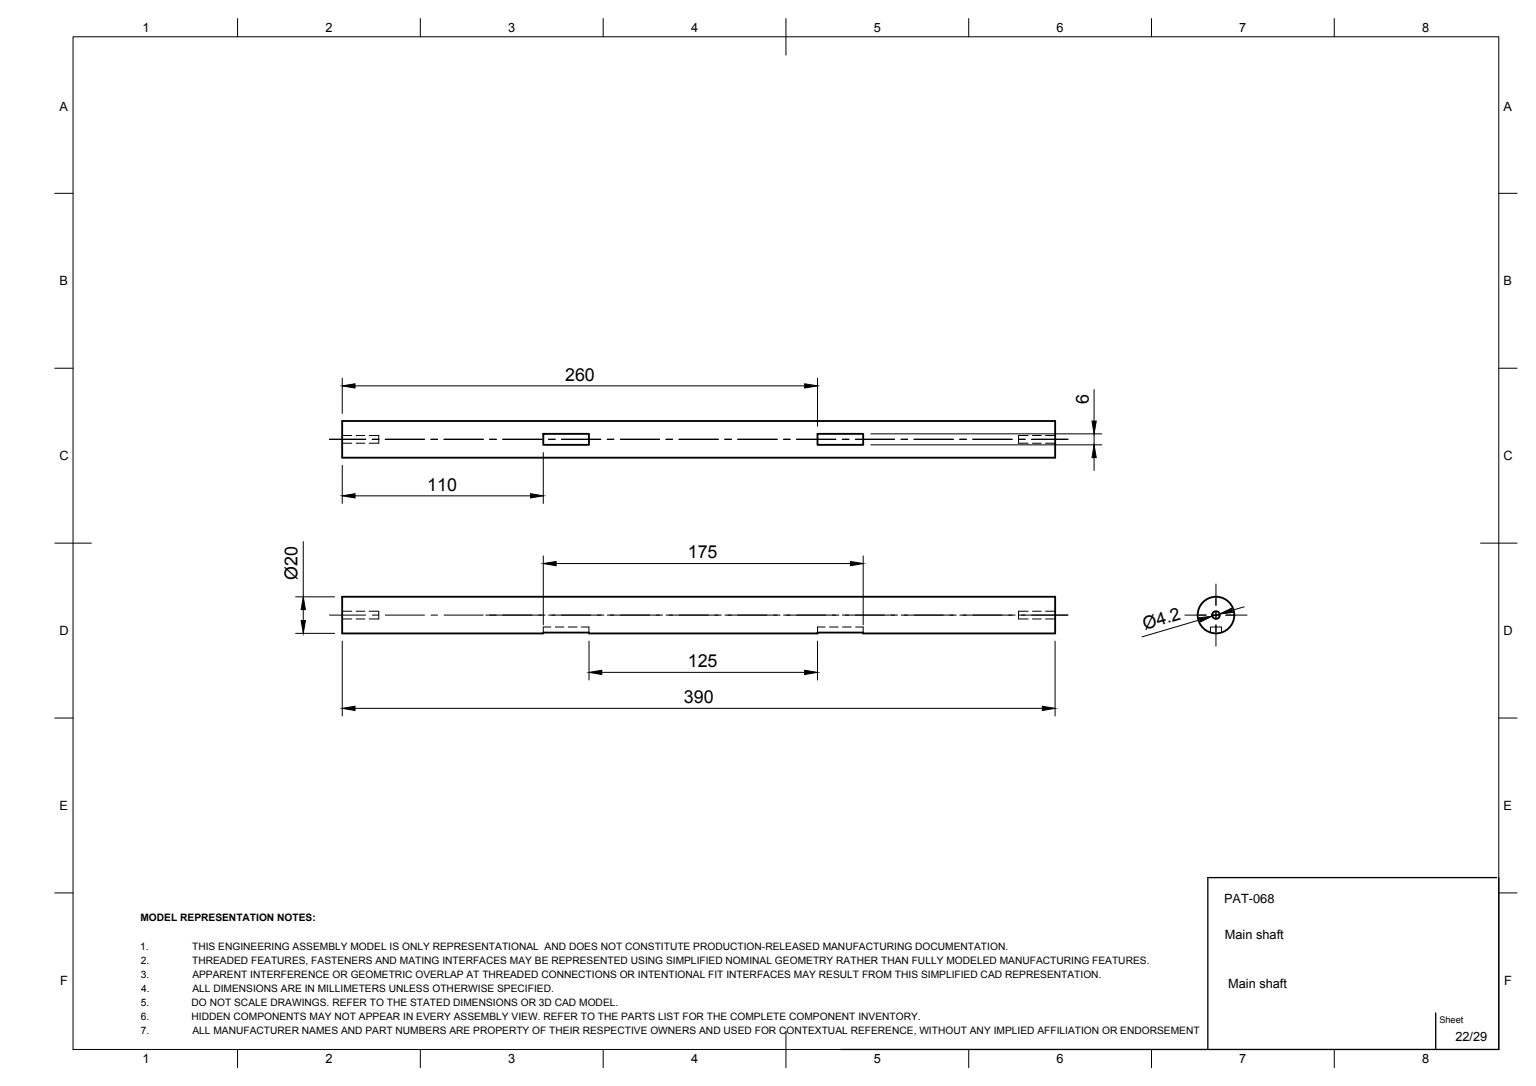
ISO-10303-21;
HEADER;
/* Generated by software containing ST-Developer
 * from STEP Tools, Inc. (www.steptools.com) 
 */

FILE_DESCRIPTION(
/* description */ ('Line shaft on three pillow blocks'),
/* implementation_level */ '2;1');

FILE_NAME(
/* name */ 'Main shaft.step',
/* time_stamp */ '2026-10-27T10:49:19-07:00',
/* author */ (''),
/* organization */ (''),
/* preprocessor_version */ 'ST-DEVELOPER v20.2',
/* originating_system */ 'Autodesk Translation Framework v15.17.0.0',
/* authorisation */ '');

FILE_SCHEMA (('AUTOMOTIVE_DESIGN { 1 0 10303 214 3 1 1 }'));
ENDSEC;

DATA;
#10=MECHANICAL_DESIGN_GEOMETRIC_PRESENTATION_REPRESENTATION('',(#356),#8377);
#301=SHAPE_REPRESENTATION_RELATIONSHIP('SRR','None',#8518,#328);
#328=ADVANCED_BREP_SHAPE_REPRESENTATION('',(#382),#8367);
#356=STYLED_ITEM('',(#8718),#382);
#382=MANIFOLD_SOLID_BREP('Body1',#4344);
#462=FACE_BOUND('',#1146,.T.);
#463=FACE_BOUND('',#1147,.T.);
#464=FACE_BOUND('',#1149,.T.);
#465=FACE_BOUND('',#1151,.T.);
#584=PLANE('',#4969);
#585=PLANE('',#4973);
#586=PLANE('',#4974);
#587=PLANE('',#4975);
#588=PLANE('',#4977);
#589=PLANE('',#4978);
#590=PLANE('',#4979);
#591=PLANE('',#4981);
#592=PLANE('',#4982);
#593=PLANE('',#4984);
#594=PLANE('',#4985);
#595=PLANE('',#4986);
#596=PLANE('',#4991);
#597=PLANE('',#4992);
#808=FACE_OUTER_BOUND('',#1131,.T.);
#809=FACE_OUTER_BOUND('',#1132,.T.);
#810=FACE_OUTER_BOUND('',#1133,.T.);
#811=FACE_OUTER_BOUND('',#1134,.T.);
#812=FACE_OUTER_BOUND('',#1135,.T.);
#813=FACE_OUTER_BOUND('',#1136,.T.);
#814=FACE_OUTER_BOUND('',#1137,.T.);
#815=FACE_OUTER_BOUND('',#1138,.T.);
#816=FACE_OUTER_BOUND('',#1139,.T.);
#817=FACE_OUTER_BOUND('',#1140,.T.);
#818=FACE_OUTER_BOUND('',#1141,.T.);
#819=FACE_OUTER_BOUND('',#1142,.T.);
#820=FACE_OUTER_BOUND('',#1143,.T.);
#821=FACE_OUTER_BOUND('',#1144,.T.);
#822=FACE_OUTER_BOUND('',#1145,.T.);
#823=FACE_OUTER_BOUND('',#1148,.T.);
#824=FACE_OUTER_BOUND('',#1150,.T.);
#1131=EDGE_LOOP('',(#3585,#3586,#3587,#3588));
#1132=EDGE_LOOP('',(#3589));
#1133=EDGE_LOOP('',(#3590,#3591,#3592,#3593));
#1134=EDGE_LOOP('',(#3594));
#1135=EDGE_LOOP('',(#3595,#3596,#3597,#3598));
#1136=EDGE_LOOP('',(#3599,#3600,#3601,#3602));
#1137=EDGE_LOOP('',(#3603,#3604,#3605,#3606));
#1138=EDGE_LOOP('',(#3607,#3608,#3609,#3610));
#1139=EDGE_LOOP('',(#3611,#3612,#3613,#3614));
#1140=EDGE_LOOP('',(#3615,#3616,#3617,#3618));
#1141=EDGE_LOOP('',(#3619,#3620,#3621,#3622));
#1142=EDGE_LOOP('',(#3623,#3624,#3625,#3626));
#1143=EDGE_LOOP('',(#3627,#3628,#3629,#3630));
#1144=EDGE_LOOP('',(#3631,#3632,#3633,#3634));
#1145=EDGE_LOOP('',(#3635,#3636,#3637,#3638));
#1146=EDGE_LOOP('',(#3639,#3640,#3641,#3642));
#1147=EDGE_LOOP('',(#3643,#3644,#3645,#3646));
#1148=EDGE_LOOP('',(#3647));
#1149=EDGE_LOOP('',(#3648));
#1150=EDGE_LOOP('',(#3649));
#1151=EDGE_LOOP('',(#3650));
#1448=LINE('',#7624,#1775);
#1449=LINE('',#7631,#1776);
#1450=LINE('',#7637,#1777);
#1451=LINE('',#7639,#1778);
#1452=LINE('',#7641,#1779);
#1453=LINE('',#7642,#1780);
#1454=LINE('',#7647,#1781);
#1455=LINE('',#7648,#1782);
#1456=LINE('',#7651,#1783);
#1457=LINE('',#7653,#1784);
#1458=LINE('',#7654,#1785);
#1459=LINE('',#7656,#1786);
#1460=LINE('',#7662,#1787);
#1461=LINE('',#7664,#1788);
#1462=LINE('',#7666,#1789);
#1463=LINE('',#7667,#1790);
#1464=LINE('',#7672,#1791);
#1465=LINE('',#7673,#1792);
#1466=LINE('',#7676,#1793);
#1467=LINE('',#7678,#1794);
#1468=LINE('',#7679,#1795);
#1469=LINE('',#7681,#1796);
#1470=LINE('',#7688,#1797);
#1775=VECTOR('',#5971,0.21);
#1776=VECTOR('',#5980,0.21);
#1777=VECTOR('',#5987,1.);
#1778=VECTOR('',#5988,1.);
#1779=VECTOR('',#5989,1.);
#1780=VECTOR('',#5990,1.);
#1781=VECTOR('',#5995,1.);
#1782=VECTOR('',#5996,1.);
#1783=VECTOR('',#5999,1.);
#1784=VECTOR('',#6000,1.);
#1785=VECTOR('',#6001,1.);
#1786=VECTOR('',#6004,1.);
#1787=VECTOR('',#6011,1.);
#1788=VECTOR('',#6012,1.);
#1789=VECTOR('',#6013,1.);
#1790=VECTOR('',#6014,1.);
#1791=VECTOR('',#6019,1.);
#1792=VECTOR('',#6020,1.);
#1793=VECTOR('',#6023,1.);
#1794=VECTOR('',#6024,1.);
#1795=VECTOR('',#6025,1.);
#1796=VECTOR('',#6028,1.);
#1797=VECTOR('',#6037,1.);
#2010=CIRCLE('',#4967,0.21);
#2011=CIRCLE('',#4968,0.21);
#2012=CIRCLE('',#4971,0.21);
#2013=CIRCLE('',#4972,0.21);
#2014=CIRCLE('',#4976,1.);
#2015=CIRCLE('',#4980,1.);
#2016=CIRCLE('',#4983,1.);
#2017=CIRCLE('',#4987,1.);
#2018=CIRCLE('',#4989,1.);
#2019=CIRCLE('',#4990,1.);
#2285=VERTEX_POINT('',#7621);
#2286=VERTEX_POINT('',#7623);
#2287=VERTEX_POINT('',#7628);
#2288=VERTEX_POINT('',#7630);
#2289=VERTEX_POINT('',#7635);
#2290=VERTEX_POINT('',#7636);
#2291=VERTEX_POINT('',#7638);
#2292=VERTEX_POINT('',#7640);
#2293=VERTEX_POINT('',#7644);
#2294=VERTEX_POINT('',#7646);
#2295=VERTEX_POINT('',#7650);
#2296=VERTEX_POINT('',#7652);
#2297=VERTEX_POINT('',#7660);
#2298=VERTEX_POINT('',#7661);
#2299=VERTEX_POINT('',#7663);
#2300=VERTEX_POINT('',#7665);
#2301=VERTEX_POINT('',#7669);
#2302=VERTEX_POINT('',#7671);
#2303=VERTEX_POINT('',#7675);
#2304=VERTEX_POINT('',#7677);
#2305=VERTEX_POINT('',#7685);
#2306=VERTEX_POINT('',#7687);
#2741=EDGE_CURVE('',#2285,#2285,#2010,.T.);
#2742=EDGE_CURVE('',#2285,#2286,#1448,.T.);
#2743=EDGE_CURVE('',#2286,#2286,#2011,.T.);
#2744=EDGE_CURVE('',#2287,#2287,#2012,.T.);
#2745=EDGE_CURVE('',#2287,#2288,#1449,.T.);
#2746=EDGE_CURVE('',#2288,#2288,#2013,.T.);
#2747=EDGE_CURVE('',#2289,#2290,#1450,.T.);
#2748=EDGE_CURVE('',#2289,#2291,#1451,.T.);
#2749=EDGE_CURVE('',#2292,#2291,#1452,.T.);
#2750=EDGE_CURVE('',#2292,#2290,#1453,.T.);
#2751=EDGE_CURVE('',#2290,#2293,#2014,.T.);
#2752=EDGE_CURVE('',#2294,#2292,#1454,.T.);
#2753=EDGE_CURVE('',#2293,#2294,#1455,.T.);
#2754=EDGE_CURVE('',#2293,#2295,#1456,.T.);
#2755=EDGE_CURVE('',#2294,#2296,#1457,.T.);
#2756=EDGE_CURVE('',#2296,#2295,#1458,.T.);
#2757=EDGE_CURVE('',#2291,#2296,#1459,.T.);
#2758=EDGE_CURVE('',#2295,#2289,#2015,.T.);
#2759=EDGE_CURVE('',#2297,#2298,#1460,.T.);
#2760=EDGE_CURVE('',#2297,#2299,#1461,.T.);
#2761=EDGE_CURVE('',#2300,#2299,#1462,.T.);
#2762=EDGE_CURVE('',#2300,#2298,#1463,.T.);
#2763=EDGE_CURVE('',#2298,#2301,#2016,.T.);
#2764=EDGE_CURVE('',#2302,#2300,#1464,.T.);
#2765=EDGE_CURVE('',#2301,#2302,#1465,.T.);
#2766=EDGE_CURVE('',#2301,#2303,#1466,.T.);
#2767=EDGE_CURVE('',#2302,#2304,#1467,.T.);
#2768=EDGE_CURVE('',#2304,#2303,#1468,.T.);
#2769=EDGE_CURVE('',#2299,#2304,#1469,.T.);
#2770=EDGE_CURVE('',#2303,#2297,#2017,.T.);
#2771=EDGE_CURVE('',#2305,#2305,#2018,.T.);
#2772=EDGE_CURVE('',#2305,#2306,#1470,.T.);
#2773=EDGE_CURVE('',#2306,#2306,#2019,.T.);
#3585=ORIENTED_EDGE('',*,*,#2741,.F.);
#3586=ORIENTED_EDGE('',*,*,#2742,.T.);
#3587=ORIENTED_EDGE('',*,*,#2743,.F.);
#3588=ORIENTED_EDGE('',*,*,#2742,.F.);
#3589=ORIENTED_EDGE('',*,*,#2741,.T.);
#3590=ORIENTED_EDGE('',*,*,#2744,.F.);
#3591=ORIENTED_EDGE('',*,*,#2745,.T.);
#3592=ORIENTED_EDGE('',*,*,#2746,.T.);
#3593=ORIENTED_EDGE('',*,*,#2745,.F.);
#3594=ORIENTED_EDGE('',*,*,#2746,.F.);
#3595=ORIENTED_EDGE('',*,*,#2747,.F.);
#3596=ORIENTED_EDGE('',*,*,#2748,.T.);
#3597=ORIENTED_EDGE('',*,*,#2749,.F.);
#3598=ORIENTED_EDGE('',*,*,#2750,.T.);
#3599=ORIENTED_EDGE('',*,*,#2751,.F.);
#3600=ORIENTED_EDGE('',*,*,#2750,.F.);
#3601=ORIENTED_EDGE('',*,*,#2752,.F.);
#3602=ORIENTED_EDGE('',*,*,#2753,.F.);
#3603=ORIENTED_EDGE('',*,*,#2754,.F.);
#3604=ORIENTED_EDGE('',*,*,#2753,.T.);
#3605=ORIENTED_EDGE('',*,*,#2755,.T.);
#3606=ORIENTED_EDGE('',*,*,#2756,.T.);
#3607=ORIENTED_EDGE('',*,*,#2752,.T.);
#3608=ORIENTED_EDGE('',*,*,#2749,.T.);
#3609=ORIENTED_EDGE('',*,*,#2757,.T.);
#3610=ORIENTED_EDGE('',*,*,#2755,.F.);
#3611=ORIENTED_EDGE('',*,*,#2758,.F.);
#3612=ORIENTED_EDGE('',*,*,#2756,.F.);
#3613=ORIENTED_EDGE('',*,*,#2757,.F.);
#3614=ORIENTED_EDGE('',*,*,#2748,.F.);
#3615=ORIENTED_EDGE('',*,*,#2759,.F.);
#3616=ORIENTED_EDGE('',*,*,#2760,.T.);
#3617=ORIENTED_EDGE('',*,*,#2761,.F.);
#3618=ORIENTED_EDGE('',*,*,#2762,.T.);
#3619=ORIENTED_EDGE('',*,*,#2763,.F.);
#3620=ORIENTED_EDGE('',*,*,#2762,.F.);
#3621=ORIENTED_EDGE('',*,*,#2764,.F.);
#3622=ORIENTED_EDGE('',*,*,#2765,.F.);
#3623=ORIENTED_EDGE('',*,*,#2766,.F.);
#3624=ORIENTED_EDGE('',*,*,#2765,.T.);
#3625=ORIENTED_EDGE('',*,*,#2767,.T.);
#3626=ORIENTED_EDGE('',*,*,#2768,.T.);
#3627=ORIENTED_EDGE('',*,*,#2764,.T.);
#3628=ORIENTED_EDGE('',*,*,#2761,.T.);
#3629=ORIENTED_EDGE('',*,*,#2769,.T.);
#3630=ORIENTED_EDGE('',*,*,#2767,.F.);
#3631=ORIENTED_EDGE('',*,*,#2770,.F.);
#3632=ORIENTED_EDGE('',*,*,#2768,.F.);
#3633=ORIENTED_EDGE('',*,*,#2769,.F.);
#3634=ORIENTED_EDGE('',*,*,#2760,.F.);
#3635=ORIENTED_EDGE('',*,*,#2771,.F.);
#3636=ORIENTED_EDGE('',*,*,#2772,.T.);
#3637=ORIENTED_EDGE('',*,*,#2773,.T.);
#3638=ORIENTED_EDGE('',*,*,#2772,.F.);
#3639=ORIENTED_EDGE('',*,*,#2754,.T.);
#3640=ORIENTED_EDGE('',*,*,#2758,.T.);
#3641=ORIENTED_EDGE('',*,*,#2747,.T.);
#3642=ORIENTED_EDGE('',*,*,#2751,.T.);
#3643=ORIENTED_EDGE('',*,*,#2766,.T.);
#3644=ORIENTED_EDGE('',*,*,#2770,.T.);
#3645=ORIENTED_EDGE('',*,*,#2759,.T.);
#3646=ORIENTED_EDGE('',*,*,#2763,.T.);
#3647=ORIENTED_EDGE('',*,*,#2771,.T.);
#3648=ORIENTED_EDGE('',*,*,#2743,.T.);
#3649=ORIENTED_EDGE('',*,*,#2773,.F.);
#3650=ORIENTED_EDGE('',*,*,#2744,.T.);
#4050=CYLINDRICAL_SURFACE('',#4966,0.21);
#4051=CYLINDRICAL_SURFACE('',#4970,0.21);
#4052=CYLINDRICAL_SURFACE('',#4988,1.);
#4226=ADVANCED_FACE('',(#808),#4050,.F.);
#4227=ADVANCED_FACE('',(#809),#584,.T.);
#4228=ADVANCED_FACE('',(#810),#4051,.F.);
#4229=ADVANCED_FACE('',(#811),#585,.F.);
#4230=ADVANCED_FACE('',(#812),#586,.F.);
#4231=ADVANCED_FACE('',(#813),#587,.T.);
#4232=ADVANCED_FACE('',(#814),#588,.F.);
#4233=ADVANCED_FACE('',(#815),#589,.F.);
#4234=ADVANCED_FACE('',(#816),#590,.F.);
#4235=ADVANCED_FACE('',(#817),#591,.F.);
#4236=ADVANCED_FACE('',(#818),#592,.T.);
#4237=ADVANCED_FACE('',(#819),#593,.F.);
#4238=ADVANCED_FACE('',(#820),#594,.F.);
#4239=ADVANCED_FACE('',(#821),#595,.F.);
#4240=ADVANCED_FACE('',(#822,#462,#463),#4052,.T.);
#4241=ADVANCED_FACE('',(#823,#464),#596,.T.);
#4242=ADVANCED_FACE('',(#824,#465),#597,.F.);
#4344=CLOSED_SHELL('',(#4226,#4227,#4228,#4229,#4230,#4231,#4232,#4233,
#4234,#4235,#4236,#4237,#4238,#4239,#4240,#4241,#4242));
#4965=AXIS2_PLACEMENT_3D('',#7619,#5965,#5966);
#4966=AXIS2_PLACEMENT_3D('',#7620,#5967,#5968);
#4967=AXIS2_PLACEMENT_3D('',#7622,#5969,#5970);
#4968=AXIS2_PLACEMENT_3D('',#7625,#5972,#5973);
#4969=AXIS2_PLACEMENT_3D('',#7626,#5974,#5975);
#4970=AXIS2_PLACEMENT_3D('',#7627,#5976,#5977);
#4971=AXIS2_PLACEMENT_3D('',#7629,#5978,#5979);
#4972=AXIS2_PLACEMENT_3D('',#7632,#5981,#5982);
#4973=AXIS2_PLACEMENT_3D('',#7633,#5983,#5984);
#4974=AXIS2_PLACEMENT_3D('',#7634,#5985,#5986);
#4975=AXIS2_PLACEMENT_3D('',#7643,#5991,#5992);
#4976=AXIS2_PLACEMENT_3D('',#7645,#5993,#5994);
#4977=AXIS2_PLACEMENT_3D('',#7649,#5997,#5998);
#4978=AXIS2_PLACEMENT_3D('',#7655,#6002,#6003);
#4979=AXIS2_PLACEMENT_3D('',#7657,#6005,#6006);
#4980=AXIS2_PLACEMENT_3D('',#7658,#6007,#6008);
#4981=AXIS2_PLACEMENT_3D('',#7659,#6009,#6010);
#4982=AXIS2_PLACEMENT_3D('',#7668,#6015,#6016);
#4983=AXIS2_PLACEMENT_3D('',#7670,#6017,#6018);
#4984=AXIS2_PLACEMENT_3D('',#7674,#6021,#6022);
#4985=AXIS2_PLACEMENT_3D('',#7680,#6026,#6027);
#4986=AXIS2_PLACEMENT_3D('',#7682,#6029,#6030);
#4987=AXIS2_PLACEMENT_3D('',#7683,#6031,#6032);
#4988=AXIS2_PLACEMENT_3D('',#7684,#6033,#6034);
#4989=AXIS2_PLACEMENT_3D('',#7686,#6035,#6036);
#4990=AXIS2_PLACEMENT_3D('',#7689,#6038,#6039);
#4991=AXIS2_PLACEMENT_3D('',#7690,#6040,#6041);
#4992=AXIS2_PLACEMENT_3D('',#7691,#6042,#6043);
#5965=DIRECTION('axis',(0.,0.,1.));
#5966=DIRECTION('refdir',(1.,0.,0.));
#5967=DIRECTION('center_axis',(0.,1.,0.));
#5968=DIRECTION('ref_axis',(1.,0.,0.));
#5969=DIRECTION('center_axis',(0.,1.,0.));
#5970=DIRECTION('ref_axis',(1.,0.,0.));
#5971=DIRECTION('',(0.,1.,0.));
#5972=DIRECTION('center_axis',(0.,-1.,0.));
#5973=DIRECTION('ref_axis',(1.,0.,0.));
#5974=DIRECTION('center_axis',(0.,1.,0.));
#5975=DIRECTION('ref_axis',(1.,0.,0.));
#5976=DIRECTION('center_axis',(0.,1.,0.));
#5977=DIRECTION('ref_axis',(1.,0.,0.));
#5978=DIRECTION('center_axis',(0.,1.,0.));
#5979=DIRECTION('ref_axis',(1.,0.,0.));
#5980=DIRECTION('',(0.,1.,0.));
#5981=DIRECTION('center_axis',(0.,1.,0.));
#5982=DIRECTION('ref_axis',(1.,0.,0.));
#5983=DIRECTION('center_axis',(0.,1.,0.));
#5984=DIRECTION('ref_axis',(1.,0.,0.));
#5985=DIRECTION('center_axis',(-1.,0.,0.));
#5986=DIRECTION('ref_axis',(0.,0.,1.));
#5987=DIRECTION('',(0.,-1.,0.));
#5988=DIRECTION('',(0.,0.,1.));
#5989=DIRECTION('',(0.,1.,0.));
#5990=DIRECTION('',(0.,0.,-1.));
#5991=DIRECTION('center_axis',(0.,1.,0.));
#5992=DIRECTION('ref_axis',(1.,0.,0.));
#5993=DIRECTION('center_axis',(0.,-1.,0.));
#5994=DIRECTION('ref_axis',(1.,0.,0.));
#5995=DIRECTION('',(-1.,0.,0.));
#5996=DIRECTION('',(0.,0.,1.));
#5997=DIRECTION('center_axis',(1.,0.,0.));
#5998=DIRECTION('ref_axis',(0.,0.,-1.));
#5999=DIRECTION('',(0.,1.,0.));
#6000=DIRECTION('',(0.,1.,0.));
#6001=DIRECTION('',(0.,0.,-1.));
#6002=DIRECTION('center_axis',(0.,0.,1.));
#6003=DIRECTION('ref_axis',(1.,0.,0.));
#6004=DIRECTION('',(1.,0.,0.));
#6005=DIRECTION('center_axis',(0.,1.,0.));
#6006=DIRECTION('ref_axis',(0.,0.,1.));
#6007=DIRECTION('center_axis',(0.,1.,0.));
#6008=DIRECTION('ref_axis',(1.,0.,0.));
#6009=DIRECTION('center_axis',(-1.,0.,0.));
#6010=DIRECTION('ref_axis',(0.,0.,1.));
#6011=DIRECTION('',(0.,-1.,0.));
#6012=DIRECTION('',(0.,0.,1.));
#6013=DIRECTION('',(0.,1.,0.));
#6014=DIRECTION('',(0.,0.,-1.));
#6015=DIRECTION('center_axis',(0.,1.,0.));
#6016=DIRECTION('ref_axis',(1.,0.,0.));
#6017=DIRECTION('center_axis',(0.,-1.,0.));
#6018=DIRECTION('ref_axis',(1.,0.,0.));
#6019=DIRECTION('',(-1.,0.,0.));
#6020=DIRECTION('',(0.,0.,1.));
#6021=DIRECTION('center_axis',(1.,0.,0.));
#6022=DIRECTION('ref_axis',(0.,0.,-1.));
#6023=DIRECTION('',(0.,1.,0.));
#6024=DIRECTION('',(0.,1.,0.));
#6025=DIRECTION('',(0.,0.,-1.));
#6026=DIRECTION('center_axis',(0.,0.,1.));
#6027=DIRECTION('ref_axis',(1.,0.,0.));
#6028=DIRECTION('',(1.,0.,0.));
#6029=DIRECTION('center_axis',(0.,1.,0.));
#6030=DIRECTION('ref_axis',(0.,0.,1.));
#6031=DIRECTION('center_axis',(0.,1.,0.));
#6032=DIRECTION('ref_axis',(1.,0.,0.));
#6033=DIRECTION('center_axis',(0.,1.,0.));
#6034=DIRECTION('ref_axis',(1.,0.,0.));
#6035=DIRECTION('center_axis',(0.,1.,0.));
#6036=DIRECTION('ref_axis',(1.,0.,0.));
#6037=DIRECTION('',(0.,-1.,0.));
#6038=DIRECTION('center_axis',(0.,1.,0.));
#6039=DIRECTION('ref_axis',(1.,0.,0.));
#6040=DIRECTION('center_axis',(0.,1.,0.));
#6041=DIRECTION('ref_axis',(1.,0.,0.));
#6042=DIRECTION('center_axis',(0.,1.,0.));
#6043=DIRECTION('ref_axis',(1.,0.,0.));
#7619=CARTESIAN_POINT('',(0.,0.,0.));
#7620=CARTESIAN_POINT('Origin',(0.,32.5,4.53));
#7621=CARTESIAN_POINT('',(-0.21,32.5,4.53));
#7622=CARTESIAN_POINT('Origin',(0.,32.5,4.53));
#7623=CARTESIAN_POINT('',(-0.21,34.5,4.53));
#7624=CARTESIAN_POINT('',(-0.21,32.5,4.53));
#7625=CARTESIAN_POINT('Origin',(0.,34.5,4.53));
#7626=CARTESIAN_POINT('Origin',(0.,32.5,4.53));
#7627=CARTESIAN_POINT('Origin',(0.,-4.6,4.53));
#7628=CARTESIAN_POINT('',(-0.21,-4.5,4.53));
#7629=CARTESIAN_POINT('Origin',(0.,-4.5,4.53));
#7630=CARTESIAN_POINT('',(-0.21,-2.5,4.53));
#7631=CARTESIAN_POINT('',(-0.21,-4.6,4.53));
#7632=CARTESIAN_POINT('Origin',(0.,-2.5,4.53));
#7633=CARTESIAN_POINT('Origin',(0.,-2.5,4.53));
#7634=CARTESIAN_POINT('Origin',(-0.3,21.,3.4));
#7635=CARTESIAN_POINT('',(-0.3,23.5,3.57606079858305));
#7636=CARTESIAN_POINT('',(-0.3,21.,3.57606079858305));
#7637=CARTESIAN_POINT('',(-0.3,-4.5,3.57606079858305));
#7638=CARTESIAN_POINT('',(-0.3,23.5,3.88));
#7639=CARTESIAN_POINT('',(-0.3,23.5,3.88));
#7640=CARTESIAN_POINT('',(-0.3,21.,3.88));
#7641=CARTESIAN_POINT('',(-0.3,21.,3.88));
#7642=CARTESIAN_POINT('',(-0.3,21.,3.88));
#7643=CARTESIAN_POINT('Origin',(0.,21.,3.64));
#7644=CARTESIAN_POINT('',(0.3,21.,3.57606079858305));
#7645=CARTESIAN_POINT('Origin',(0.,21.,4.53));
#7646=CARTESIAN_POINT('',(0.3,21.,3.88));
#7647=CARTESIAN_POINT('',(0.3,21.,3.88));
#7648=CARTESIAN_POINT('',(0.3,21.,3.4));
#7649=CARTESIAN_POINT('Origin',(0.3,21.,3.88));
#7650=CARTESIAN_POINT('',(0.3,23.5,3.57606079858305));
#7651=CARTESIAN_POINT('',(0.3,-4.5,3.57606079858305));
#7652=CARTESIAN_POINT('',(0.3,23.5,3.88));
#7653=CARTESIAN_POINT('',(0.3,21.,3.88));
#7654=CARTESIAN_POINT('',(0.3,23.5,3.4));
#7655=CARTESIAN_POINT('Origin',(-0.3,21.,3.88));
#7656=CARTESIAN_POINT('',(0.3,23.5,3.88));
#7657=CARTESIAN_POINT('Origin',(0.,23.5,3.64));
#7658=CARTESIAN_POINT('Origin',(0.,23.5,4.53));
#7659=CARTESIAN_POINT('Origin',(-0.3,6.,3.4));
#7660=CARTESIAN_POINT('',(-0.3,8.5,3.57606079858305));
#7661=CARTESIAN_POINT('',(-0.3,6.,3.57606079858305));
#7662=CARTESIAN_POINT('',(-0.3,-4.5,3.57606079858305));
#7663=CARTESIAN_POINT('',(-0.3,8.5,3.88));
#7664=CARTESIAN_POINT('',(-0.3,8.5,3.88));
#7665=CARTESIAN_POINT('',(-0.3,6.,3.88));
#7666=CARTESIAN_POINT('',(-0.3,6.,3.88));
#7667=CARTESIAN_POINT('',(-0.3,6.,3.88));
#7668=CARTESIAN_POINT('Origin',(0.,6.,3.64));
#7669=CARTESIAN_POINT('',(0.3,6.,3.57606079858305));
#7670=CARTESIAN_POINT('Origin',(0.,6.,4.53));
#7671=CARTESIAN_POINT('',(0.3,6.,3.88));
#7672=CARTESIAN_POINT('',(0.3,6.,3.88));
#7673=CARTESIAN_POINT('',(0.3,6.,3.4));
#7674=CARTESIAN_POINT('Origin',(0.3,6.,3.88));
#7675=CARTESIAN_POINT('',(0.3,8.5,3.57606079858305));
#7676=CARTESIAN_POINT('',(0.3,-4.5,3.57606079858305));
#7677=CARTESIAN_POINT('',(0.3,8.5,3.88));
#7678=CARTESIAN_POINT('',(0.3,6.,3.88));
#7679=CARTESIAN_POINT('',(0.3,8.5,3.4));
#7680=CARTESIAN_POINT('Origin',(-0.3,6.,3.88));
#7681=CARTESIAN_POINT('',(0.3,8.5,3.88));
#7682=CARTESIAN_POINT('Origin',(0.,8.5,3.64));
#7683=CARTESIAN_POINT('Origin',(0.,8.5,4.53));
#7684=CARTESIAN_POINT('Origin',(0.,-4.5,4.53));
#7685=CARTESIAN_POINT('',(-1.,34.5,4.53));
#7686=CARTESIAN_POINT('Origin',(0.,34.5,4.53));
#7687=CARTESIAN_POINT('',(-1.,-4.5,4.53));
#7688=CARTESIAN_POINT('',(-1.,-4.5,4.53));
#7689=CARTESIAN_POINT('Origin',(0.,-4.5,4.53));
#7690=CARTESIAN_POINT('Origin',(0.,34.5,4.53));
#7691=CARTESIAN_POINT('Origin',(0.,-4.5,4.53));
#8335=UNCERTAINTY_MEASURE_WITH_UNIT(LENGTH_MEASURE(0.001),#8378,
'DISTANCE_ACCURACY_VALUE',
'Maximum model space distance between geometric entities at asserted c
onnectivities');
#8345=UNCERTAINTY_MEASURE_WITH_UNIT(LENGTH_MEASURE(0.001),#8378,
'DISTANCE_ACCURACY_VALUE',
'Maximum model space distance between geometric entities at asserted c
onnectivities');
#8367=(
GEOMETRIC_REPRESENTATION_CONTEXT(3)
GLOBAL_UNCERTAINTY_ASSIGNED_CONTEXT((#8335))
GLOBAL_UNIT_ASSIGNED_CONTEXT((#8378,#8380,#8381))
REPRESENTATION_CONTEXT('','3D')
);
#8377=(
GEOMETRIC_REPRESENTATION_CONTEXT(3)
GLOBAL_UNCERTAINTY_ASSIGNED_CONTEXT((#8345))
GLOBAL_UNIT_ASSIGNED_CONTEXT((#8378,#8380,#8381))
REPRESENTATION_CONTEXT('','3D')
);
#8378=(
LENGTH_UNIT()
NAMED_UNIT(*)
SI_UNIT(.CENTI.,.METRE.)
);
#8380=(
NAMED_UNIT(*)
PLANE_ANGLE_UNIT()
SI_UNIT($,.RADIAN.)
);
#8381=(
NAMED_UNIT(*)
SI_UNIT($,.STERADIAN.)
SOLID_ANGLE_UNIT()
);
#8403=SHAPE_DEFINITION_REPRESENTATION(#8470,#8518);
#8470=PRODUCT_DEFINITION_SHAPE('',$,#8550);
#8518=SHAPE_REPRESENTATION('',(#4965),#8367);
#8528=PRODUCT_DEFINITION_CONTEXT('part definition',#8623,'design');
#8550=PRODUCT_DEFINITION('Main shaft','Main shaft',#8581,#8528);
#8581=PRODUCT_DEFINITION_FORMATION('',$,#8646);
#8623=APPLICATION_CONTEXT(
'Core Data for Automotive Mechanical Design Process');
#8624=PRODUCT_CONTEXT('part definition',#8623,'mechanical');
#8646=PRODUCT('Main shaft','Main shaft','Main shaft',(#8624));
#8712=COLOUR_RGB('Grey',0.48,0.52,0.57);
#8713=FILL_AREA_STYLE_COLOUR('',#8712);
#8714=FILL_AREA_STYLE('',(#8713));
#8715=SURFACE_STYLE_FILL_AREA(#8714);
#8716=SURFACE_SIDE_STYLE('',(#8715));
#8717=SURFACE_STYLE_USAGE(.BOTH.,#8716);
#8718=PRESENTATION_STYLE_ASSIGNMENT((#8717));
ENDSEC;
END-ISO-10303-21;
